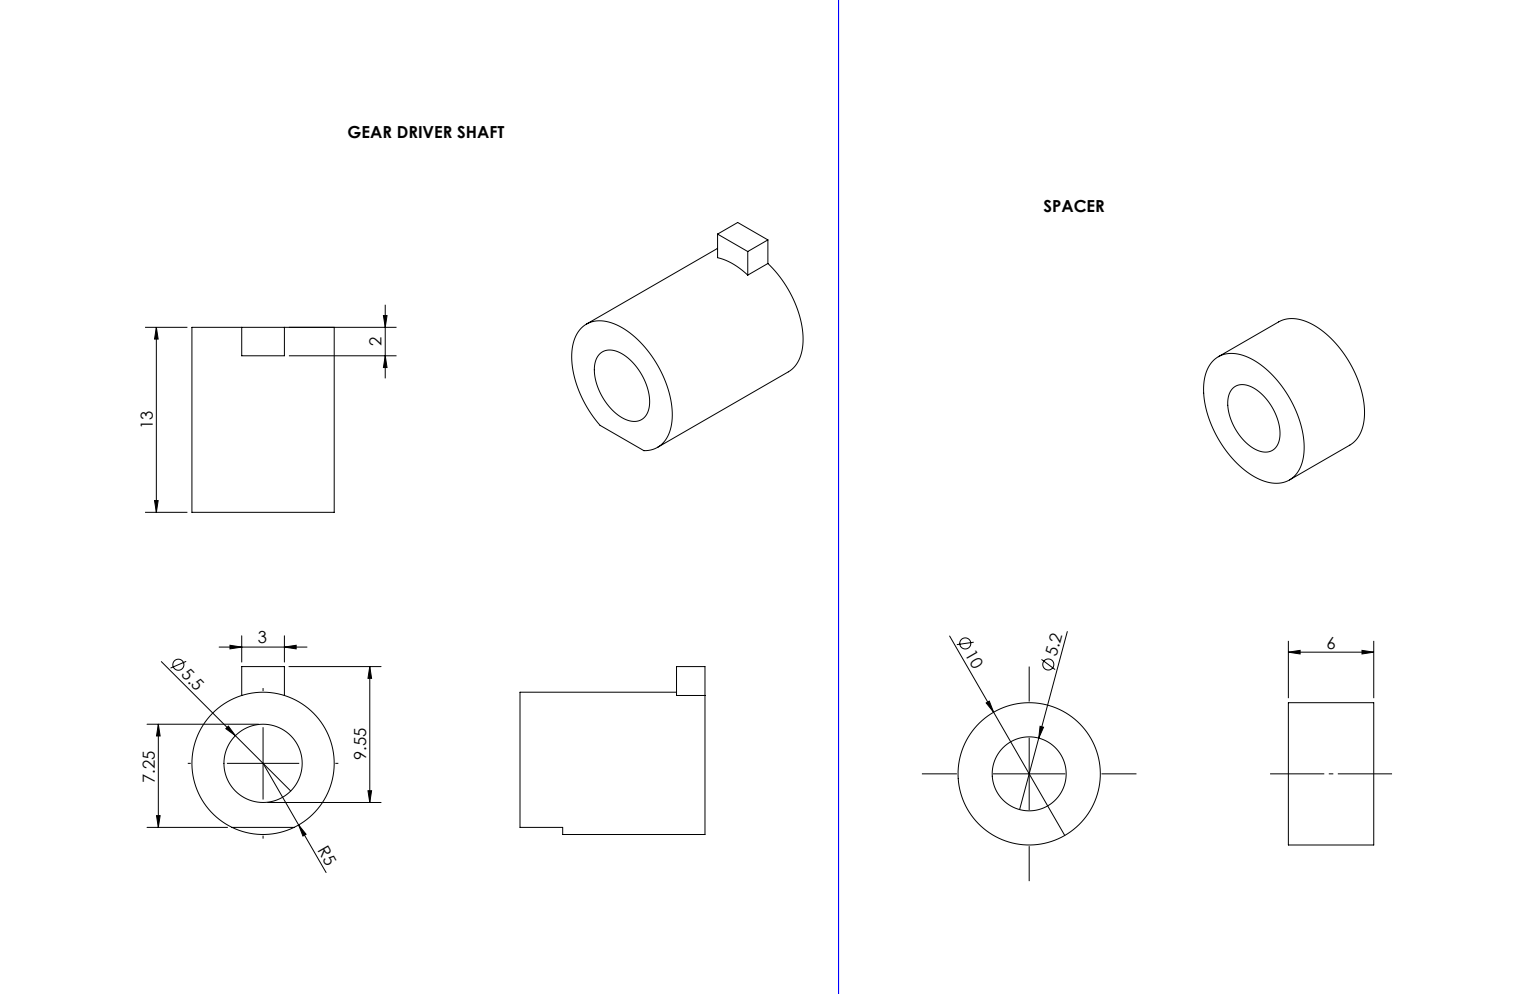
ISO-10303-21;
HEADER;
FILE_DESCRIPTION (('STEP AP214'),
    '1' );
FILE_NAME ('gear driver shaft.step',
    '2026-09-24T10:15:42',
    ( '' ),
    ( '' ),
    'SwSTEP 2.0',
    'SolidWorks 2026',
    '' );
FILE_SCHEMA (( 'AUTOMOTIVE_DESIGN' ));
ENDSEC;

DATA;
#66=LINE ( 'NONE', #18792, #4083 ) ;
#134=AXIS2_PLACEMENT_3D ( 'NONE', #17909, #414, #1850 ) ;
#150=VECTOR ( 'NONE', #10844, 1000.000000000000000 ) ;
#156=ORIENTED_EDGE ( 'NONE', *, *, #8866, .F. ) ;
#178=( GEOMETRIC_REPRESENTATION_CONTEXT ( 3 ) GLOBAL_UNCERTAINTY_ASSIGNED_CONTEXT ( ( #14166 ) ) GLOBAL_UNIT_ASSIGNED_CONTEXT ( ( #7797, #12606, #6360 ) ) REPRESENTATION_CONTEXT ( 'NONE', 'WORKASPACE' ) );
#246=EDGE_CURVE ( 'NONE', #12932, #11930, #3616, .T. ) ;
#414=DIRECTION ( 'NONE',  ( -0.000000000000000000, -0.000000000000000000, 1.000000000000000000 ) ) ;
#429=DIRECTION ( 'NONE',  ( 1.000000000000000000, 1.913297951445007868E-16, -0.000000000000000000 ) ) ;
#446=ORIENTED_EDGE ( 'NONE', *, *, #4582, .F. ) ;
#572=EDGE_LOOP ( 'NONE', ( #726, #446 ) ) ;
#576=CARTESIAN_POINT ( 'NONE',  ( 0.000000000000000000, 0.000000000000000000, -3.000000000000000000 ) ) ;
#577=CARTESIAN_POINT ( 'NONE',  ( 2.749999999999996891, 0.000000000000000000, -6.000000000000000888 ) ) ;
#613=CIRCLE ( 'NONE', #11582, 5.000000000000000000 ) ;
#726=ORIENTED_EDGE ( 'NONE', *, *, #6443, .F. ) ;
#782=AXIS2_PLACEMENT_3D ( 'NONE', #11547, #18892, #1309 ) ;
#819=VERTEX_POINT ( 'NONE', #14412 ) ;
#893=EDGE_CURVE ( 'NONE', #11930, #15939, #2932, .T. ) ;
#908=ORIENTED_EDGE ( 'NONE', *, *, #17596, .T. ) ;
#931=DIRECTION ( 'NONE',  ( -0.000000000000000000, -0.000000000000000000, 1.000000000000000000 ) ) ;
#978=VERTEX_POINT ( 'NONE', #4488 ) ;
#995=ORIENTED_EDGE ( 'NONE', *, *, #893, .T. ) ;
#1043=CARTESIAN_POINT ( 'NONE',  ( 2.749999999999997335, 0.000000000000000000, 7.000000000000000000 ) ) ;
#1108=ADVANCED_FACE ( 'NONE', ( #11167 ), #6399, .F. ) ;
#1142=SURFACE_STYLE_FILL_AREA ( #6542 ) ;
#1158=DIRECTION ( 'NONE',  ( -1.000000000000000000, 0.000000000000000000, 0.000000000000000000 ) ) ;
#1199=CARTESIAN_POINT ( 'NONE',  ( 1.499999999999999112, 4.769696007084728073, 5.000000000000000000 ) ) ;
#1240=ADVANCED_BREP_SHAPE_REPRESENTATION ( '', ( #9885, #2030 ), #4780 ) ;
#1292=CARTESIAN_POINT ( 'NONE',  ( -1.500000000000001332, 6.799999999999999822, 7.000000000000000000 ) ) ;
#1309=DIRECTION ( 'NONE',  ( 1.000000000000000000, 0.000000000000000000, 0.000000000000000000 ) ) ;
#1381=VECTOR ( 'NONE', #12196, 1000.000000000000000 ) ;
#1382=FACE_OUTER_BOUND ( 'NONE', #10839, .T. ) ;
#1478=ADVANCED_FACE ( 'NONE', ( #18646 ), #18461, .F. ) ;
#1497=ORIENTED_EDGE ( 'NONE', *, *, #5425, .T. ) ;
#1502=ORIENTED_EDGE ( 'NONE', *, *, #17596, .F. ) ;
#1521=ORIENTED_EDGE ( 'NONE', *, *, #16735, .T. ) ;
#1526=ORIENTED_EDGE ( 'NONE', *, *, #4878, .F. ) ;
#1551=SURFACE_SIDE_STYLE ('',( #10249 ) ) ;
#1632=ORIENTED_EDGE ( 'NONE', *, *, #246, .T. ) ;
#1640=VECTOR ( 'NONE', #17756, 1000.000000000000000 ) ;
#1788=PLANE ( 'NONE',  #4428 ) ;
#1793=CARTESIAN_POINT ( 'NONE',  ( 0.000000000000000000, 0.000000000000000000, -3.000000000000000000 ) ) ;
#1850=DIRECTION ( 'NONE',  ( 1.000000000000000000, 0.000000000000000000, 0.000000000000000000 ) ) ;
#1881=EDGE_LOOP ( 'NONE', ( #8452, #16560, #5178, #17650, #3158, #7094, #9920, #7769 ) ) ;
#1971=CIRCLE ( 'NONE', #3477, 5.000000000000000000 ) ;
#2009=LINE ( 'NONE', #7558, #8984 ) ;
#2030=AXIS2_PLACEMENT_3D ( 'NONE', #15716, #11248, #17249 ) ;
#2095=AXIS2_PLACEMENT_3D ( 'NONE', #13304, #6051, #11878 ) ;
#2205=VECTOR ( 'NONE', #1158, 1000.000000000000000 ) ;
#2273=PLANE ( 'NONE',  #9044 ) ;
#2366=ORIENTED_EDGE ( 'NONE', *, *, #3270, .T. ) ;
#2487=FACE_OUTER_BOUND ( 'NONE', #15895, .T. ) ;
#2497=SHAPE_DEFINITION_REPRESENTATION ( #4797, #12894 ) ;
#2564=DIRECTION ( 'NONE',  ( 1.000000000000000000, 0.000000000000000000, 0.000000000000000000 ) ) ;
#2675=DIRECTION ( 'NONE',  ( 0.000000000000000000, -0.000000000000000000, 1.000000000000000000 ) ) ;
#2704=EDGE_CURVE ( 'NONE', #12932, #11277, #12193, .T. ) ;
#2776=FILL_AREA_STYLE ('',( #7593 ) ) ;
#2804=EDGE_CURVE ( 'NONE', #2807, #819, #7009, .T. ) ;
#2807=VERTEX_POINT ( 'NONE', #6022 ) ;
#2890=CARTESIAN_POINT ( 'NONE',  ( 0.000000000000000000, 0.000000000000000000, -3.000000000000000000 ) ) ;
#2925=ORIENTED_EDGE ( 'NONE', *, *, #18359, .F. ) ;
#2932=LINE ( 'NONE', #9923, #14944 ) ;
#3080=UNCERTAINTY_MEASURE_WITH_UNIT (LENGTH_MEASURE( 1.000000000000000082E-05 ), #13302, 'distance_accuracy_value', 'NONE');
#3082=LINE ( 'NONE', #15996, #9638 ) ;
#3158=ORIENTED_EDGE ( 'NONE', *, *, #4711, .F. ) ;
#3165=EDGE_LOOP ( 'NONE', ( #13969, #1526, #1502, #12720 ) ) ;
#3168=EDGE_LOOP ( 'NONE', ( #3631, #18900, #4290, #7846 ) ) ;
#3192=EDGE_CURVE ( 'NONE', #978, #9121, #613, .T. ) ;
#3270=EDGE_CURVE ( 'NONE', #8048, #14890, #5993, .T. ) ;
#3309=DIRECTION ( 'NONE',  ( -0.000000000000000000, -0.000000000000000000, -1.000000000000000000 ) ) ;
#3398=DIRECTION ( 'NONE',  ( 1.000000000000000000, 1.913297951445007868E-16, -0.000000000000000000 ) ) ;
#3401=DIRECTION ( 'NONE',  ( 1.000000000000000000, 0.000000000000000000, 0.000000000000000000 ) ) ;
#3477=AXIS2_PLACEMENT_3D ( 'NONE', #1793, #7634, #3401 ) ;
#3503=PRODUCT_DEFINITION_CONTEXT ( 'detailed design', #7680, 'design' ) ;
#3616=CIRCLE ( 'NONE', #6058, 5.000000000000000000 ) ;
#3631=ORIENTED_EDGE ( 'NONE', *, *, #14197, .F. ) ;
#3853=CARTESIAN_POINT ( 'NONE',  ( -1.500000000000001332, 6.799999999999999822, 5.000000000000000000 ) ) ;
#3900=EDGE_LOOP ( 'NONE', ( #5999, #4562 ) ) ;
#3911=ORIENTED_EDGE ( 'NONE', *, *, #14218, .F. ) ;
#3942=DIRECTION ( 'NONE',  ( 0.000000000000000000, 1.000000000000000000, 0.000000000000000000 ) ) ;
#4016=CARTESIAN_POINT ( 'NONE',  ( 0.000000000000000000, 0.000000000000000000, 7.000000000000000000 ) ) ;
#4023=ORIENTED_EDGE ( 'NONE', *, *, #18359, .T. ) ;
#4043=CARTESIAN_POINT ( 'NONE',  ( -1.500000000000000888, 4.769696007084728073, -3.000000000000000000 ) ) ;
#4048=CYLINDRICAL_SURFACE ( 'NONE', #7572, 2.749999999999997335 ) ;
#4083=VECTOR ( 'NONE', #8661, 1000.000000000000000 ) ;
#4128=PLANE ( 'NONE',  #14182 ) ;
#4170=ORIENTED_EDGE ( 'NONE', *, *, #11302, .F. ) ;
#4192=CARTESIAN_POINT ( 'NONE',  ( 1.499999999999998668, 6.799999999999999822, 5.000000000000000000 ) ) ;
#4248=VERTEX_POINT ( 'NONE', #10411 ) ;
#4257=VECTOR ( 'NONE', #3309, 1000.000000000000000 ) ;
#4269=ORIENTED_EDGE ( 'NONE', *, *, #14784, .F. ) ;
#4290=ORIENTED_EDGE ( 'NONE', *, *, #7556, .T. ) ;
#4301=DIRECTION ( 'NONE',  ( -0.000000000000000000, -0.000000000000000000, 1.000000000000000000 ) ) ;
#4339=ORIENTED_EDGE ( 'NONE', *, *, #10048, .F. ) ;
#4352=CARTESIAN_POINT ( 'NONE',  ( 1.499999999999998668, 6.799999999999999822, 7.000000000000000000 ) ) ;
#4428=AXIS2_PLACEMENT_3D ( 'NONE', #4750, #3398, #9235 ) ;
#4474=MECHANICAL_DESIGN_GEOMETRIC_PRESENTATION_REPRESENTATION('',(#15448),#15756);
#4488=CARTESIAN_POINT ( 'NONE',  ( -1.500000000000000888, 4.769696007084728073, 7.000000000000000000 ) ) ;
#4517=EDGE_CURVE ( 'NONE', #4248, #9121, #66, .T. ) ;
#4522=AXIS2_PLACEMENT_3D ( 'NONE', #4617, #14358, #16084 ) ;
#4562=ORIENTED_EDGE ( 'NONE', *, *, #14197, .T. ) ;
#4567=CARTESIAN_POINT ( 'NONE',  ( 1.499999999999999112, 4.769696007084728073, -3.000000000000000000 ) ) ;
#4582=EDGE_CURVE ( 'NONE', #9014, #7450, #1971, .T. ) ;
#4617=CARTESIAN_POINT ( 'NONE',  ( 0.000000000000000000, 0.000000000000000000, -6.000000000000000000 ) ) ;
#4637=FACE_OUTER_BOUND ( 'NONE', #1881, .T. ) ;
#4711=EDGE_CURVE ( 'NONE', #11930, #7450, #14880, .T. ) ;
#4750=CARTESIAN_POINT ( 'NONE',  ( -1.500000000000000000, -2.869946927167511679E-16, 5.000000000000000000 ) ) ;
#4767=ORIENTED_EDGE ( 'NONE', *, *, #7354, .F. ) ;
#4780=( GEOMETRIC_REPRESENTATION_CONTEXT ( 3 ) GLOBAL_UNCERTAINTY_ASSIGNED_CONTEXT ( ( #3080 ) ) GLOBAL_UNIT_ASSIGNED_CONTEXT ( ( #13302, #13017, #8903 ) ) REPRESENTATION_CONTEXT ( 'NONE', 'WORKASPACE' ) );
#4797=PRODUCT_DEFINITION_SHAPE ( 'NONE', 'NONE',  #5434 ) ;
#4848=FACE_OUTER_BOUND ( 'NONE', #17818, .T. ) ;
#4878=EDGE_CURVE ( 'NONE', #10634, #13856, #2009, .T. ) ;
#4921=FACE_OUTER_BOUND ( 'NONE', #16434, .T. ) ;
#4977=VECTOR ( 'NONE', #15693, 1000.000000000000000 ) ;
#4998=ORIENTED_EDGE ( 'NONE', *, *, #18182, .F. ) ;
#5001=CARTESIAN_POINT ( 'NONE',  ( -2.179449471770337432, -4.500000000000000000, -6.000000000000000000 ) ) ;
#5118=EDGE_CURVE ( 'NONE', #7783, #12607, #18145, .T. ) ;
#5142=DIRECTION ( 'NONE',  ( 0.000000000000000000, 0.000000000000000000, 1.000000000000000000 ) ) ;
#5178=ORIENTED_EDGE ( 'NONE', *, *, #7354, .T. ) ;
#5219=ADVANCED_FACE ( 'NONE', ( #16839 ), #9485, .T. ) ;
#5250=DIRECTION ( 'NONE',  ( -0.000000000000000000, -0.000000000000000000, 1.000000000000000000 ) ) ;
#5255=DIRECTION ( 'NONE',  ( 1.000000000000000000, 0.000000000000000000, 0.000000000000000000 ) ) ;
#5313=DIRECTION ( 'NONE',  ( 1.000000000000000000, 0.000000000000000000, 0.000000000000000000 ) ) ;
#5338=ORIENTED_EDGE ( 'NONE', *, *, #7986, .F. ) ;
#5375=DIRECTION ( 'NONE',  ( 1.000000000000000000, 0.000000000000000000, 0.000000000000000000 ) ) ;
#5413=ORIENTED_EDGE ( 'NONE', *, *, #4711, .T. ) ;
#5425=EDGE_CURVE ( 'NONE', #15939, #4248, #5683, .T. ) ;
#5434=PRODUCT_DEFINITION ( 'UNKNOWN', '', #13558, #3503 ) ;
#5614=DIRECTION ( 'NONE',  ( -0.000000000000000000, -0.000000000000000000, 1.000000000000000000 ) ) ;
#5683=CIRCLE ( 'NONE', #15470, 5.000000000000000000 ) ;
#5740=( NAMED_UNIT ( * ) PLANE_ANGLE_UNIT ( ) SI_UNIT ( $, .RADIAN. ) );
#5766=DIRECTION ( 'NONE',  ( 1.000000000000000000, 0.000000000000000000, 0.000000000000000000 ) ) ;
#5962=UNCERTAINTY_MEASURE_WITH_UNIT (LENGTH_MEASURE( 1.000000000000000082E-05 ), #7202, 'distance_accuracy_value', 'NONE');
#5963=COLOUR_RGB ( '', 0.72549020, 0.75294118, 0.79215686) ;
#5980=ORIENTED_EDGE ( 'NONE', *, *, #16025, .T. ) ;
#5993=LINE ( 'NONE', #4567, #4257 ) ;
#5999=ORIENTED_EDGE ( 'NONE', *, *, #5118, .T. ) ;
#6022=CARTESIAN_POINT ( 'NONE',  ( -1.500000000000001332, 6.799999999999999822, 5.000000000000000000 ) ) ;
#6042=ORIENTED_EDGE ( 'NONE', *, *, #3192, .T. ) ;
#6051=DIRECTION ( 'NONE',  ( -0.000000000000000000, -0.000000000000000000, 1.000000000000000000 ) ) ;
#6058=AXIS2_PLACEMENT_3D ( 'NONE', #10555, #16387, #17727 ) ;
#6287=CARTESIAN_POINT ( 'NONE',  ( 2.179449471770337432, -4.500000000000000000, -6.000000000000000000 ) ) ;
#6314=CARTESIAN_POINT ( 'NONE',  ( 0.000000000000000000, 0.000000000000000000, -6.000000000000000000 ) ) ;
#6358=LINE ( 'NONE', #5001, #150 ) ;
#6360=( NAMED_UNIT ( * ) SI_UNIT ( $, .STERADIAN. ) SOLID_ANGLE_UNIT ( ) );
#6399=PLANE ( 'NONE',  #7166 ) ;
#6443=EDGE_CURVE ( 'NONE', #7450, #9014, #18835, .T. ) ;
#6467=ADVANCED_FACE ( 'NONE', ( #7090 ), #12908, .F. ) ;
#6542=FILL_AREA_STYLE ('',( #10748 ) ) ;
#6588=FACE_OUTER_BOUND ( 'NONE', #6729, .T. ) ;
#6643=CARTESIAN_POINT ( 'NONE',  ( -1.500000000000000000, -2.869946927167511679E-16, 7.000000000000000000 ) ) ;
#6695=APPLICATION_CONTEXT ( 'automotive_design' ) ;
#6719=DIRECTION ( 'NONE',  ( -1.000000000000000000, 0.000000000000000000, -0.000000000000000000 ) ) ;
#6729=EDGE_LOOP ( 'NONE', ( #6042, #7134, #8063, #8870, #4269, #13753 ) ) ;
#6817=DIRECTION ( 'NONE',  ( 1.000000000000000000, 0.000000000000000000, 0.000000000000000000 ) ) ;
#6844=AXIS2_PLACEMENT_3D ( 'NONE', #12261, #9394, #6719 ) ;
#6905=CARTESIAN_POINT ( 'NONE',  ( 2.179449471770337432, -4.500000000000000000, -6.000000000000000000 ) ) ;
#6968=DIRECTION ( 'NONE',  ( 1.000000000000000000, 0.000000000000000000, 0.000000000000000000 ) ) ;
#6986=SURFACE_SIDE_STYLE ('',( #1142 ) ) ;
#6995=CARTESIAN_POINT ( 'NONE',  ( -2.749999999999996891, 3.367778697655217067E-16, -6.000000000000000888 ) ) ;
#7009=LINE ( 'NONE', #3853, #11501 ) ;
#7016=CARTESIAN_POINT ( 'NONE',  ( 0.000000000000000000, 0.000000000000000000, -6.000000000000000888 ) ) ;
#7090=FACE_OUTER_BOUND ( 'NONE', #3165, .T. ) ;
#7094=ORIENTED_EDGE ( 'NONE', *, *, #246, .F. ) ;
#7134=ORIENTED_EDGE ( 'NONE', *, *, #18587, .T. ) ;
#7166=AXIS2_PLACEMENT_3D ( 'NONE', #576, #5142, #15453 ) ;
#7202=( LENGTH_UNIT ( ) NAMED_UNIT ( * ) SI_UNIT ( .MILLI., .METRE. ) );
#7226=CARTESIAN_POINT ( 'NONE',  ( -2.749999999999997780, 3.367778697655218546E-16, 7.000000000000000000 ) ) ;
#7286=DIRECTION ( 'NONE',  ( 0.000000000000000000, -1.000000000000000000, 0.000000000000000000 ) ) ;
#7322=DIRECTION ( 'NONE',  ( -1.913297951445007622E-16, 1.000000000000000000, 0.000000000000000000 ) ) ;
#7354=EDGE_CURVE ( 'NONE', #15939, #9014, #6358, .T. ) ;
#7393=( NAMED_UNIT ( * ) SI_UNIT ( $, .STERADIAN. ) SOLID_ANGLE_UNIT ( ) );
#7446=ADVANCED_FACE ( 'NONE', ( #2487 ), #4128, .F. ) ;
#7450=VERTEX_POINT ( 'NONE', #15589 ) ;
#7493=AXIS2_PLACEMENT_3D ( 'NONE', #12365, #15508, #6817 ) ;
#7515=AXIS2_PLACEMENT_3D ( 'NONE', #6314, #13182, #7662 ) ;
#7525=ORIENTED_EDGE ( 'NONE', *, *, #17215, .T. ) ;
#7556=EDGE_CURVE ( 'NONE', #17875, #11285, #8104, .T. ) ;
#7558=CARTESIAN_POINT ( 'NONE',  ( 1.499999999999998668, 6.799999999999999822, 5.000000000000000000 ) ) ;
#7572=AXIS2_PLACEMENT_3D ( 'NONE', #15697, #8443, #11413 ) ;
#7593=FILL_AREA_STYLE_COLOUR ( '', #10906 ) ;
#7634=DIRECTION ( 'NONE',  ( 0.000000000000000000, 0.000000000000000000, 1.000000000000000000 ) ) ;
#7662=DIRECTION ( 'NONE',  ( 1.000000000000000000, 0.000000000000000000, 0.000000000000000000 ) ) ;
#7665=CARTESIAN_POINT ( 'NONE',  ( 2.179449471770337432, -4.500000000000000000, -6.000000000000000000 ) ) ;
#7680=APPLICATION_CONTEXT ( 'automotive_design' ) ;
#7760=ORIENTED_EDGE ( 'NONE', *, *, #4517, .T. ) ;
#7769=ORIENTED_EDGE ( 'NONE', *, *, #18587, .F. ) ;
#7783=VERTEX_POINT ( 'NONE', #577 ) ;
#7797=( LENGTH_UNIT ( ) NAMED_UNIT ( * ) SI_UNIT ( .MILLI., .METRE. ) );
#7846=ORIENTED_EDGE ( 'NONE', *, *, #17215, .F. ) ;
#7906=LINE ( 'NONE', #16679, #1381 ) ;
#7986=EDGE_CURVE ( 'NONE', #12607, #17875, #8206, .T. ) ;
#7990=LINE ( 'NONE', #6643, #11612 ) ;
#8048=VERTEX_POINT ( 'NONE', #13347 ) ;
#8063=ORIENTED_EDGE ( 'NONE', *, *, #18182, .T. ) ;
#8071=ORIENTED_EDGE ( 'NONE', *, *, #16025, .F. ) ;
#8104=CIRCLE ( 'NONE', #17235, 2.749999999999998224 ) ;
#8114=ADVANCED_FACE ( 'NONE', ( #4848 ), #1788, .F. ) ;
#8174=PRODUCT_CONTEXT ( 'NONE', #6695, 'mechanical' ) ;
#8175=LINE ( 'NONE', #4043, #4977 ) ;
#8206=LINE ( 'NONE', #14027, #12664 ) ;
#8411=MECHANICAL_DESIGN_GEOMETRIC_PRESENTATION_REPRESENTATION('',(#12079),#178);
#8422=CARTESIAN_POINT ( 'NONE',  ( -1.500000000000001332, 6.799999999999999822, 5.000000000000000000 ) ) ;
#8443=DIRECTION ( 'NONE',  ( -0.000000000000000000, -0.000000000000000000, 1.000000000000000000 ) ) ;
#8452=ORIENTED_EDGE ( 'NONE', *, *, #4517, .F. ) ;
#8486=ADVANCED_FACE ( 'NONE', ( #12583, #6588 ), #2273, .T. ) ;
#8661=DIRECTION ( 'NONE',  ( 0.000000000000000000, 0.000000000000000000, 1.000000000000000000 ) ) ;
#8663=CARTESIAN_POINT ( 'NONE',  ( 5.000000000000000000, 0.000000000000000000, -6.000000000000000000 ) ) ;
#8860=CARTESIAN_POINT ( 'NONE',  ( 0.000000000000000000, 0.000000000000000000, 7.000000000000000000 ) ) ;
#8866=EDGE_CURVE ( 'NONE', #8048, #13856, #15257, .T. ) ;
#8870=ORIENTED_EDGE ( 'NONE', *, *, #8866, .T. ) ;
#8903=( NAMED_UNIT ( * ) SI_UNIT ( $, .STERADIAN. ) SOLID_ANGLE_UNIT ( ) );
#8984=VECTOR ( 'NONE', #17684, 1000.000000000000000 ) ;
#9002=CIRCLE ( 'NONE', #13587, 5.000000000000000000 ) ;
#9006=ORIENTED_EDGE ( 'NONE', *, *, #10230, .F. ) ;
#9014=VERTEX_POINT ( 'NONE', #13134 ) ;
#9044=AXIS2_PLACEMENT_3D ( 'NONE', #16721, #14029, #15632 ) ;
#9071=CLOSED_SHELL ( 'NONE', ( #1478, #17903, #1108, #9170, #8486, #16694, #8114, #6467, #5219, #7446, #14241, #15318 ) ) ;
#9121=VERTEX_POINT ( 'NONE', #17828 ) ;
#9162=ORIENTED_EDGE ( 'NONE', *, *, #10230, .T. ) ;
#9170=ADVANCED_FACE ( 'NONE', ( #4637 ), #14949, .T. ) ;
#9176=AXIS2_PLACEMENT_3D ( 'NONE', #10751, #429, #11993 ) ;
#9234=DIRECTION ( 'NONE',  ( -0.000000000000000000, -0.000000000000000000, 1.000000000000000000 ) ) ;
#9235=DIRECTION ( 'NONE',  ( -1.913297951445007868E-16, 1.000000000000000000, 0.000000000000000000 ) ) ;
#9243=DIRECTION ( 'NONE',  ( 1.000000000000000000, 0.000000000000000000, 0.000000000000000000 ) ) ;
#9316=DIRECTION ( 'NONE',  ( 0.000000000000000000, 0.000000000000000000, 1.000000000000000000 ) ) ;
#9355=ORIENTED_EDGE ( 'NONE', *, *, #14218, .T. ) ;
#9394=DIRECTION ( 'NONE',  ( 0.000000000000000000, 0.000000000000000000, -1.000000000000000000 ) ) ;
#9485=PLANE ( 'NONE',  #6844 ) ;
#9584=DIRECTION ( 'NONE',  ( -1.913297951445007622E-16, 1.000000000000000000, 0.000000000000000000 ) ) ;
#9591=DIRECTION ( 'NONE',  ( -0.000000000000000000, -0.000000000000000000, 1.000000000000000000 ) ) ;
#9596=ORIENTED_EDGE ( 'NONE', *, *, #7556, .F. ) ;
#9638=VECTOR ( 'NONE', #7322, 1000.000000000000000 ) ;
#9663=CIRCLE ( 'NONE', #11207, 5.000000000000000000 ) ;
#9667=CARTESIAN_POINT ( 'NONE',  ( 0.000000000000000000, 0.000000000000000000, -6.000000000000000000 ) ) ;
#9743=CARTESIAN_POINT ( 'NONE',  ( 0.000000000000000000, 0.000000000000000000, 7.000000000000000000 ) ) ;
#9869=EDGE_LOOP ( 'NONE', ( #3911, #9596 ) ) ;
#9885=MANIFOLD_SOLID_BREP ( 'M5 Clearance Hole1', #9071 ) ;
#9920=ORIENTED_EDGE ( 'NONE', *, *, #2704, .T. ) ;
#9923=CARTESIAN_POINT ( 'NONE',  ( 2.179449471770337432, -4.500000000000000000, -6.000000000000000000 ) ) ;
#9947=ORIENTED_EDGE ( 'NONE', *, *, #2704, .F. ) ;
#9955=DIRECTION ( 'NONE',  ( 0.000000000000000000, 0.000000000000000000, 1.000000000000000000 ) ) ;
#10040=CARTESIAN_POINT ( 'NONE',  ( 2.179449471770337432, -4.500000000000000000, -3.000000000000000000 ) ) ;
#10045=ORIENTED_EDGE ( 'NONE', *, *, #4878, .T. ) ;
#10048=EDGE_CURVE ( 'NONE', #14890, #10634, #3082, .T. ) ;
#10129=CARTESIAN_POINT ( 'NONE',  ( -1.500000000000000888, 4.769696007084728073, 5.000000000000000000 ) ) ;
#10230=EDGE_CURVE ( 'NONE', #10313, #2807, #7906, .T. ) ;
#10249=SURFACE_STYLE_FILL_AREA ( #2776 ) ;
#10313=VERTEX_POINT ( 'NONE', #10129 ) ;
#10320=CIRCLE ( 'NONE', #2095, 2.749999999999998224 ) ;
#10411=CARTESIAN_POINT ( 'NONE',  ( -5.000000000000000000, 6.123233995736766282E-16, -6.000000000000000000 ) ) ;
#10491=AXIS2_PLACEMENT_3D ( 'NONE', #14074, #9234, #5375 ) ;
#10555=CARTESIAN_POINT ( 'NONE',  ( 0.000000000000000000, 0.000000000000000000, -6.000000000000000000 ) ) ;
#10634=VERTEX_POINT ( 'NONE', #4192 ) ;
#10661=PLANE ( 'NONE',  #9176 ) ;
#10748=FILL_AREA_STYLE_COLOUR ( '', #5963 ) ;
#10751=CARTESIAN_POINT ( 'NONE',  ( 1.500000000000000000, 2.869946927167511679E-16, 5.000000000000000000 ) ) ;
#10839=EDGE_LOOP ( 'NONE', ( #2925, #7760, #18803, #17475, #8071, #16549, #4998, #9947 ) ) ;
#10844=DIRECTION ( 'NONE',  ( -0.000000000000000000, -0.000000000000000000, 1.000000000000000000 ) ) ;
#10906=COLOUR_RGB ( '', 0.72549020, 0.75294118, 0.79215686) ;
#11167=FACE_OUTER_BOUND ( 'NONE', #572, .T. ) ;
#11207=AXIS2_PLACEMENT_3D ( 'NONE', #18345, #5250, #14044 ) ;
#11248=DIRECTION ( 'NONE',  ( 0.000000000000000000, 0.000000000000000000, 1.000000000000000000 ) ) ;
#11277=VERTEX_POINT ( 'NONE', #17047 ) ;
#11285=VERTEX_POINT ( 'NONE', #13990 ) ;
#11302=EDGE_CURVE ( 'NONE', #978, #10313, #8175, .T. ) ;
#11367=ORIENTED_EDGE ( 'NONE', *, *, #10048, .T. ) ;
#11386=DIRECTION ( 'NONE',  ( -0.000000000000000000, 0.000000000000000000, -1.000000000000000000 ) ) ;
#11413=DIRECTION ( 'NONE',  ( 1.000000000000000000, 0.000000000000000000, 0.000000000000000000 ) ) ;
#11501=VECTOR ( 'NONE', #9955, 1000.000000000000000 ) ;
#11547=CARTESIAN_POINT ( 'NONE',  ( 0.000000000000000000, 0.000000000000000000, 7.000000000000000000 ) ) ;
#11582=AXIS2_PLACEMENT_3D ( 'NONE', #8860, #13159, #6968 ) ;
#11612=VECTOR ( 'NONE', #9584, 1000.000000000000000 ) ;
#11878=DIRECTION ( 'NONE',  ( 1.000000000000000000, 0.000000000000000000, 0.000000000000000000 ) ) ;
#11891=VECTOR ( 'NONE', #9243, 1000.000000000000000 ) ;
#11930=VERTEX_POINT ( 'NONE', #7665 ) ;
#11993=DIRECTION ( 'NONE',  ( -1.913297951445007868E-16, 1.000000000000000000, 0.000000000000000000 ) ) ;
#12055=CARTESIAN_POINT ( 'NONE',  ( -2.179449471770337432, -4.500000000000000000, -6.000000000000000000 ) ) ;
#12079=STYLED_ITEM ( 'NONE', ( #18622 ), #9885 ) ;
#12120=LINE ( 'NONE', #15068, #11891 ) ;
#12193=LINE ( 'NONE', #18199, #13654 ) ;
#12196=DIRECTION ( 'NONE',  ( -1.913297951445007622E-16, 1.000000000000000000, 0.000000000000000000 ) ) ;
#12261=CARTESIAN_POINT ( 'NONE',  ( 0.000000000000000000, 0.000000000000000000, 5.000000000000000000 ) ) ;
#12365=CARTESIAN_POINT ( 'NONE',  ( 0.000000000000000000, 0.000000000000000000, -3.000000000000000000 ) ) ;
#12461=AXIS2_PLACEMENT_3D ( 'NONE', #7016, #9591, #15421 ) ;
#12583=FACE_BOUND ( 'NONE', #9869, .T. ) ;
#12606=( NAMED_UNIT ( * ) PLANE_ANGLE_UNIT ( ) SI_UNIT ( $, .RADIAN. ) );
#12607=VERTEX_POINT ( 'NONE', #6995 ) ;
#12664=VECTOR ( 'NONE', #931, 1000.000000000000000 ) ;
#12720=ORIENTED_EDGE ( 'NONE', *, *, #2804, .T. ) ;
#12799=SURFACE_STYLE_USAGE ( .BOTH. , #6986 ) ;
#12815=ORIENTED_EDGE ( 'NONE', *, *, #2804, .F. ) ;
#12894=SHAPE_REPRESENTATION ( 'gear driver shaft', ( #2030 ), #4780 ) ;
#12908=PLANE ( 'NONE',  #16243 ) ;
#12932=VERTEX_POINT ( 'NONE', #8663 ) ;
#13017=( NAMED_UNIT ( * ) PLANE_ANGLE_UNIT ( ) SI_UNIT ( $, .RADIAN. ) );
#13039=DIRECTION ( 'NONE',  ( 0.000000000000000000, 0.000000000000000000, 1.000000000000000000 ) ) ;
#13134=CARTESIAN_POINT ( 'NONE',  ( -2.179449471770337432, -4.500000000000000000, -3.000000000000000000 ) ) ;
#13159=DIRECTION ( 'NONE',  ( 0.000000000000000000, 0.000000000000000000, 1.000000000000000000 ) ) ;
#13182=DIRECTION ( 'NONE',  ( -0.000000000000000000, 0.000000000000000000, -1.000000000000000000 ) ) ;
#13302=( LENGTH_UNIT ( ) NAMED_UNIT ( * ) SI_UNIT ( .MILLI., .METRE. ) );
#13304=CARTESIAN_POINT ( 'NONE',  ( 0.000000000000000000, 0.000000000000000000, 7.000000000000000000 ) ) ;
#13305=VECTOR ( 'NONE', #18218, 1000.000000000000000 ) ;
#13347=CARTESIAN_POINT ( 'NONE',  ( 1.499999999999999112, 4.769696007084728073, 7.000000000000000000 ) ) ;
#13390=ORIENTED_EDGE ( 'NONE', *, *, #5118, .F. ) ;
#13558=PRODUCT_DEFINITION_FORMATION_WITH_SPECIFIED_SOURCE ( 'ANY', '', #16234, .NOT_KNOWN. ) ;
#13587=AXIS2_PLACEMENT_3D ( 'NONE', #4016, #15666, #2564 ) ;
#13654=VECTOR ( 'NONE', #9316, 1000.000000000000000 ) ;
#13753=ORIENTED_EDGE ( 'NONE', *, *, #16735, .F. ) ;
#13856=VERTEX_POINT ( 'NONE', #4352 ) ;
#13969=ORIENTED_EDGE ( 'NONE', *, *, #14784, .T. ) ;
#13987=CIRCLE ( 'NONE', #12461, 2.749999999999996891 ) ;
#13990=CARTESIAN_POINT ( 'NONE',  ( 2.749999999999998224, 0.000000000000000000, 7.000000000000000000 ) ) ;
#14027=CARTESIAN_POINT ( 'NONE',  ( -2.749999999999997335, 3.367778697655217560E-16, 7.000000000000000000 ) ) ;
#14029=DIRECTION ( 'NONE',  ( 0.000000000000000000, 0.000000000000000000, 1.000000000000000000 ) ) ;
#14044=DIRECTION ( 'NONE',  ( -1.000000000000000000, -1.776356839400250465E-15, 0.000000000000000000 ) ) ;
#14074=CARTESIAN_POINT ( 'NONE',  ( 0.000000000000000000, 0.000000000000000000, 7.000000000000000000 ) ) ;
#14139=LINE ( 'NONE', #1043, #15878 ) ;
#14166=UNCERTAINTY_MEASURE_WITH_UNIT (LENGTH_MEASURE( 1.000000000000000082E-05 ), #7797, 'distance_accuracy_value', 'NONE');
#14182=AXIS2_PLACEMENT_3D ( 'NONE', #6905, #3942, #2675 ) ;
#14193=AXIS2_PLACEMENT_3D ( 'NONE', #2890, #13039, #5766 ) ;
#14197=EDGE_CURVE ( 'NONE', #12607, #7783, #13987, .T. ) ;
#14218=EDGE_CURVE ( 'NONE', #11285, #17875, #10320, .T. ) ;
#14241=ADVANCED_FACE ( 'NONE', ( #15979, #17717 ), #14642, .F. ) ;
#14249=VECTOR ( 'NONE', #5313, 1000.000000000000000 ) ;
#14358=DIRECTION ( 'NONE',  ( 0.000000000000000000, -0.000000000000000000, 1.000000000000000000 ) ) ;
#14412=CARTESIAN_POINT ( 'NONE',  ( -1.500000000000001332, 6.799999999999999822, 7.000000000000000000 ) ) ;
#14450=PRESENTATION_STYLE_ASSIGNMENT (( #16081 ) ) ;
#14640=SHAPE_REPRESENTATION_RELATIONSHIP ( 'NONE' , 'NONE' ,  #12894, #1240 ) ;
#14642=PLANE ( 'NONE',  #4522 ) ;
#14784=EDGE_CURVE ( 'NONE', #819, #13856, #15820, .T. ) ;
#14880=LINE ( 'NONE', #6287, #1640 ) ;
#14890=VERTEX_POINT ( 'NONE', #1199 ) ;
#14944=VECTOR ( 'NONE', #17380, 1000.000000000000000 ) ;
#14949=CYLINDRICAL_SURFACE ( 'NONE', #7493, 5.000000000000000000 ) ;
#15068=CARTESIAN_POINT ( 'NONE',  ( -1.500000000000001332, 6.799999999999999822, 5.000000000000000000 ) ) ;
#15207=EDGE_LOOP ( 'NONE', ( #5338, #13390, #7525, #9355 ) ) ;
#15257=LINE ( 'NONE', #18308, #13305 ) ;
#15318=ADVANCED_FACE ( 'NONE', ( #17137 ), #4048, .F. ) ;
#15421=DIRECTION ( 'NONE',  ( 1.000000000000000000, 0.000000000000000000, 0.000000000000000000 ) ) ;
#15435=ORIENTED_EDGE ( 'NONE', *, *, #893, .F. ) ;
#15448=STYLED_ITEM ( 'NONE', ( #14450 ), #1240 ) ;
#15453=DIRECTION ( 'NONE',  ( 1.000000000000000000, 0.000000000000000000, -0.000000000000000000 ) ) ;
#15470=AXIS2_PLACEMENT_3D ( 'NONE', #9667, #11386, #15493 ) ;
#15493=DIRECTION ( 'NONE',  ( 1.000000000000000000, 0.000000000000000000, 0.000000000000000000 ) ) ;
#15508=DIRECTION ( 'NONE',  ( 0.000000000000000000, 0.000000000000000000, 1.000000000000000000 ) ) ;
#15589=CARTESIAN_POINT ( 'NONE',  ( 2.179449471770337432, -4.500000000000000000, -3.000000000000000000 ) ) ;
#15632=DIRECTION ( 'NONE',  ( 1.000000000000000000, 0.000000000000000000, -0.000000000000000000 ) ) ;
#15666=DIRECTION ( 'NONE',  ( 0.000000000000000000, 0.000000000000000000, 1.000000000000000000 ) ) ;
#15675=DIRECTION ( 'NONE',  ( 0.000000000000000000, -0.000000000000000000, -1.000000000000000000 ) ) ;
#15693=DIRECTION ( 'NONE',  ( -0.000000000000000000, -0.000000000000000000, -1.000000000000000000 ) ) ;
#15697=CARTESIAN_POINT ( 'NONE',  ( 0.000000000000000000, 0.000000000000000000, 7.000000000000000000 ) ) ;
#15716=CARTESIAN_POINT ( 'NONE',  ( 0.000000000000000000, 0.000000000000000000, 0.000000000000000000 ) ) ;
#15756=( GEOMETRIC_REPRESENTATION_CONTEXT ( 3 ) GLOBAL_UNCERTAINTY_ASSIGNED_CONTEXT ( ( #5962 ) ) GLOBAL_UNIT_ASSIGNED_CONTEXT ( ( #7202, #5740, #7393 ) ) REPRESENTATION_CONTEXT ( 'NONE', 'WORKASPACE' ) );
#15820=LINE ( 'NONE', #1292, #14249 ) ;
#15878=VECTOR ( 'NONE', #4301, 1000.000000000000000 ) ;
#15895=EDGE_LOOP ( 'NONE', ( #16967, #4767, #15435, #5413 ) ) ;
#15939=VERTEX_POINT ( 'NONE', #12055 ) ;
#15979=FACE_BOUND ( 'NONE', #3900, .T. ) ;
#15995=CYLINDRICAL_SURFACE ( 'NONE', #14193, 5.000000000000000000 ) ;
#15996=CARTESIAN_POINT ( 'NONE',  ( 1.500000000000000000, 2.869946927167511679E-16, 5.000000000000000000 ) ) ;
#16025=EDGE_CURVE ( 'NONE', #14890, #10313, #9663, .T. ) ;
#16081=SURFACE_STYLE_USAGE ( .BOTH. , #1551 ) ;
#16084=DIRECTION ( 'NONE',  ( 1.000000000000000000, 0.000000000000000000, -0.000000000000000000 ) ) ;
#16234=PRODUCT ( 'gear driver shaft', 'gear driver shaft', '', ( #8174 ) ) ;
#16243=AXIS2_PLACEMENT_3D ( 'NONE', #8422, #7286, #15675 ) ;
#16354=CIRCLE ( 'NONE', #7515, 5.000000000000000000 ) ;
#16387=DIRECTION ( 'NONE',  ( -0.000000000000000000, 0.000000000000000000, -1.000000000000000000 ) ) ;
#16434=EDGE_LOOP ( 'NONE', ( #156, #2366, #11367, #10045 ) ) ;
#16549=ORIENTED_EDGE ( 'NONE', *, *, #3270, .F. ) ;
#16560=ORIENTED_EDGE ( 'NONE', *, *, #5425, .F. ) ;
#16679=CARTESIAN_POINT ( 'NONE',  ( -1.500000000000000000, -2.869946927167511679E-16, 5.000000000000000000 ) ) ;
#16694=ADVANCED_FACE ( 'NONE', ( #4921 ), #10661, .T. ) ;
#16721=CARTESIAN_POINT ( 'NONE',  ( 0.000000000000000000, 0.000000000000000000, 7.000000000000000000 ) ) ;
#16735=EDGE_CURVE ( 'NONE', #978, #819, #7990, .T. ) ;
#16839=FACE_OUTER_BOUND ( 'NONE', #17686, .T. ) ;
#16967=ORIENTED_EDGE ( 'NONE', *, *, #6443, .T. ) ;
#17047=CARTESIAN_POINT ( 'NONE',  ( 5.000000000000000000, 0.000000000000000000, 7.000000000000000000 ) ) ;
#17137=FACE_OUTER_BOUND ( 'NONE', #15207, .T. ) ;
#17158=EDGE_LOOP ( 'NONE', ( #1497, #4023, #1632, #995 ) ) ;
#17215=EDGE_CURVE ( 'NONE', #7783, #11285, #14139, .T. ) ;
#17235=AXIS2_PLACEMENT_3D ( 'NONE', #9743, #5614, #5255 ) ;
#17249=DIRECTION ( 'NONE',  ( 1.000000000000000000, 0.000000000000000000, 0.000000000000000000 ) ) ;
#17380=DIRECTION ( 'NONE',  ( -1.000000000000000000, 0.000000000000000000, 0.000000000000000000 ) ) ;
#17475=ORIENTED_EDGE ( 'NONE', *, *, #11302, .T. ) ;
#17596=EDGE_CURVE ( 'NONE', #2807, #10634, #12120, .T. ) ;
#17650=ORIENTED_EDGE ( 'NONE', *, *, #4582, .T. ) ;
#17684=DIRECTION ( 'NONE',  ( 0.000000000000000000, 0.000000000000000000, 1.000000000000000000 ) ) ;
#17686=EDGE_LOOP ( 'NONE', ( #4339, #5980, #9162, #908 ) ) ;
#17717=FACE_OUTER_BOUND ( 'NONE', #17158, .T. ) ;
#17727=DIRECTION ( 'NONE',  ( 1.000000000000000000, 0.000000000000000000, 0.000000000000000000 ) ) ;
#17756=DIRECTION ( 'NONE',  ( -0.000000000000000000, -0.000000000000000000, 1.000000000000000000 ) ) ;
#17818=EDGE_LOOP ( 'NONE', ( #4170, #1521, #12815, #9006 ) ) ;
#17828=CARTESIAN_POINT ( 'NONE',  ( -5.000000000000000000, 6.123233995736766282E-16, 7.000000000000000000 ) ) ;
#17875=VERTEX_POINT ( 'NONE', #7226 ) ;
#17903=ADVANCED_FACE ( 'NONE', ( #1382 ), #15995, .T. ) ;
#17909=CARTESIAN_POINT ( 'NONE',  ( 0.000000000000000000, 0.000000000000000000, -6.000000000000000888 ) ) ;
#18145=CIRCLE ( 'NONE', #134, 2.749999999999996891 ) ;
#18182=EDGE_CURVE ( 'NONE', #11277, #8048, #9002, .T. ) ;
#18199=CARTESIAN_POINT ( 'NONE',  ( 5.000000000000000000, 0.000000000000000000, -3.000000000000000000 ) ) ;
#18218=DIRECTION ( 'NONE',  ( -1.913297951445007622E-16, 1.000000000000000000, 0.000000000000000000 ) ) ;
#18308=CARTESIAN_POINT ( 'NONE',  ( 1.500000000000000000, 2.869946927167511679E-16, 7.000000000000000000 ) ) ;
#18345=CARTESIAN_POINT ( 'NONE',  ( 0.000000000000000000, 0.000000000000000000, 5.000000000000000000 ) ) ;
#18359=EDGE_CURVE ( 'NONE', #4248, #12932, #16354, .T. ) ;
#18461=CYLINDRICAL_SURFACE ( 'NONE', #10491, 2.749999999999997335 ) ;
#18587=EDGE_CURVE ( 'NONE', #9121, #11277, #18772, .T. ) ;
#18622=PRESENTATION_STYLE_ASSIGNMENT (( #12799 ) ) ;
#18646=FACE_OUTER_BOUND ( 'NONE', #3168, .T. ) ;
#18772=CIRCLE ( 'NONE', #782, 5.000000000000000000 ) ;
#18792=CARTESIAN_POINT ( 'NONE',  ( -5.000000000000000000, 6.123233995736766282E-16, -3.000000000000000000 ) ) ;
#18803=ORIENTED_EDGE ( 'NONE', *, *, #3192, .F. ) ;
#18835=LINE ( 'NONE', #10040, #2205 ) ;
#18892=DIRECTION ( 'NONE',  ( 0.000000000000000000, 0.000000000000000000, 1.000000000000000000 ) ) ;
#18900=ORIENTED_EDGE ( 'NONE', *, *, #7986, .T. ) ;
ENDSEC;
END-ISO-10303-21;
